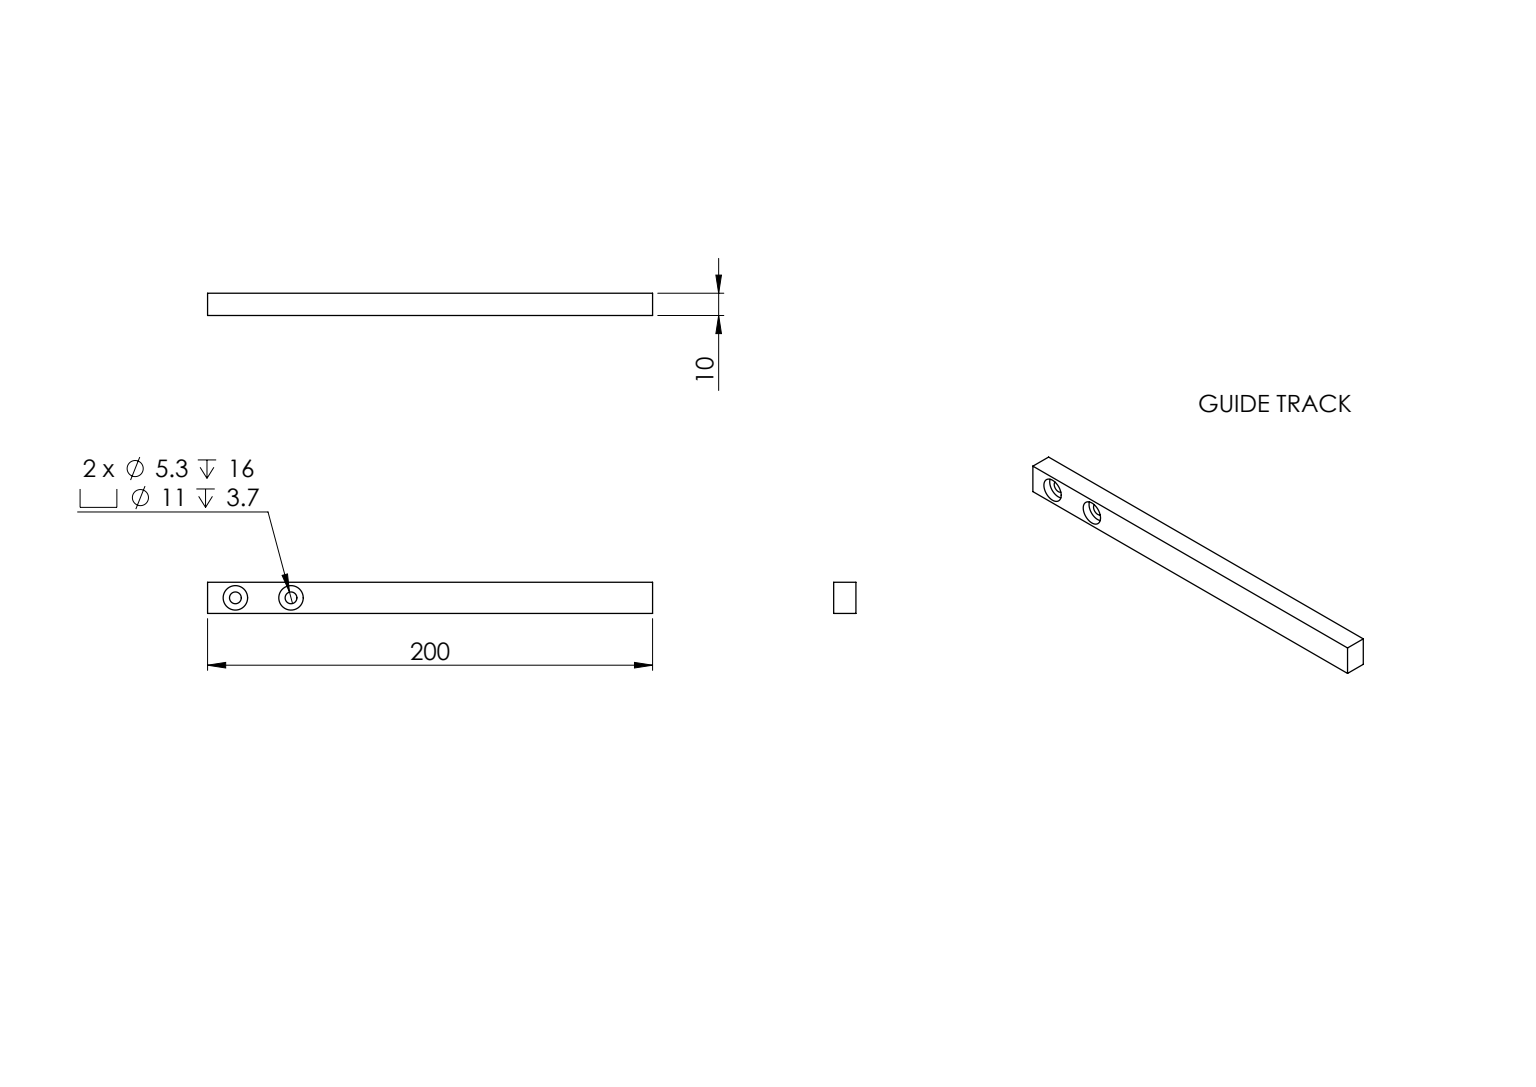
ISO-10303-21;
HEADER;
FILE_DESCRIPTION (('STEP AP214'),
    '1' );
FILE_NAME ('guide track.step',
    '2026-10-27T14:18:53',
    ( '' ),
    ( '' ),
    'SwSTEP 2.0',
    'SolidWorks 2026',
    '' );
FILE_SCHEMA (( 'AUTOMOTIVE_DESIGN' ));
ENDSEC;

DATA;
#9=CIRCLE ( 'NONE', #2713, 2.649999999999999467 ) ;
#10=FACE_OUTER_BOUND ( 'NONE', #5268, .T. ) ;
#20=ADVANCED_FACE ( 'NONE', ( #1293 ), #2022, .F. ) ;
#49=EDGE_LOOP ( 'NONE', ( #4386, #5805, #654, #4968 ) ) ;
#54=CARTESIAN_POINT ( 'NONE',  ( 0.000000000000000000, 0.000000000000000000, 75.00000000000000000 ) ) ;
#60=VERTEX_POINT ( 'NONE', #3659 ) ;
#71=AXIS2_PLACEMENT_3D ( 'NONE', #3867, #5717, #1567 ) ;
#76=CARTESIAN_POINT ( 'NONE',  ( 24.99999999999998224, 6.999999999999985789, 65.00000000000000000 ) ) ;
#84=DIRECTION ( 'NONE',  ( 0.000000000000000000, 0.000000000000000000, 1.000000000000000000 ) ) ;
#91=ADVANCED_FACE ( 'NONE', ( #3214 ), #1319, .F. ) ;
#92=ORIENTED_EDGE ( 'NONE', *, *, #3018, .T. ) ;
#95=DIRECTION ( 'NONE',  ( -0.000000000000000000, -0.000000000000000000, 1.000000000000000000 ) ) ;
#131=EDGE_CURVE ( 'NONE', #60, #666, #9, .T. ) ;
#173=DIRECTION ( 'NONE',  ( -1.000000000000000000, -0.000000000000000000, -0.000000000000000000 ) ) ;
#175=ORIENTED_EDGE ( 'NONE', *, *, #2979, .F. ) ;
#185=AXIS2_PLACEMENT_3D ( 'NONE', #3101, #5825, #5378 ) ;
#220=LINE ( 'NONE', #1177, #2270 ) ;
#235=EDGE_LOOP ( 'NONE', ( #5621, #519 ) ) ;
#242=FACE_BOUND ( 'NONE', #235, .T. ) ;
#271=CARTESIAN_POINT ( 'NONE',  ( 24.99999999999998224, 6.999999999999985789, 75.00000000000000000 ) ) ;
#310=PRESENTATION_STYLE_ASSIGNMENT (( #4469 ) ) ;
#343=CARTESIAN_POINT ( 'NONE',  ( 68.00000000000000000, -1.951563910473909559E-15, 75.00000000000000000 ) ) ;
#346=SHAPE_REPRESENTATION_RELATIONSHIP ( 'NONE' , 'NONE' ,  #2785, #5722 ) ;
#391=DIRECTION ( 'NONE',  ( -0.000000000000000000, -0.000000000000000000, 1.000000000000000000 ) ) ;
#426=CARTESIAN_POINT ( 'NONE',  ( 24.99999999999998224, 6.999999999999985789, 75.00000000000000000 ) ) ;
#438=ORIENTED_EDGE ( 'NONE', *, *, #2529, .F. ) ;
#440=EDGE_LOOP ( 'NONE', ( #5310, #2912, #92, #4963 ) ) ;
#448=EDGE_LOOP ( 'NONE', ( #5357, #973 ) ) ;
#457=DIRECTION ( 'NONE',  ( -0.000000000000000000, -0.000000000000000000, 1.000000000000000000 ) ) ;
#461=EDGE_CURVE ( 'NONE', #5479, #5285, #3793, .T. ) ;
#472=DIRECTION ( 'NONE',  ( 1.000000000000000000, 0.000000000000000000, 0.000000000000000000 ) ) ;
#487=EDGE_LOOP ( 'NONE', ( #1577, #4433, #2223, #5314 ) ) ;
#508=ORIENTED_EDGE ( 'NONE', *, *, #4349, .F. ) ;
#513=DIRECTION ( 'NONE',  ( -0.000000000000000000, -0.000000000000000000, 1.000000000000000000 ) ) ;
#519=ORIENTED_EDGE ( 'NONE', *, *, #2394, .F. ) ;
#566=DIRECTION ( 'NONE',  ( -0.000000000000000000, -0.000000000000000000, 1.000000000000000000 ) ) ;
#599=EDGE_CURVE ( 'NONE', #3899, #5382, #1521, .T. ) ;
#613=CARTESIAN_POINT ( 'NONE',  ( 57.00000000000002132, -1.278008170942866441E-15, 75.00000000000000000 ) ) ;
#615=PRODUCT_DEFINITION_FORMATION_WITH_SPECIFIED_SOURCE ( 'ANY', '', #682, .NOT_KNOWN. ) ;
#638=ORIENTED_EDGE ( 'NONE', *, *, #2527, .F. ) ;
#651=DIRECTION ( 'NONE',  ( -0.000000000000000000, -0.000000000000000000, 1.000000000000000000 ) ) ;
#654=ORIENTED_EDGE ( 'NONE', *, *, #3425, .F. ) ;
#666=VERTEX_POINT ( 'NONE', #3916 ) ;
#667=DIRECTION ( 'NONE',  ( 1.000000000000000000, 0.000000000000000000, 0.000000000000000000 ) ) ;
#681=CARTESIAN_POINT ( 'NONE',  ( 62.50000000000001421, -1.951563910473909559E-15, 75.00000000000000000 ) ) ;
#682=PRODUCT ( 'guide track', 'guide track', '', ( #3710 ) ) ;
#690=DIRECTION ( 'NONE',  ( -0.000000000000000000, -0.000000000000000000, 1.000000000000000000 ) ) ;
#693=CARTESIAN_POINT ( 'NONE',  ( 62.50000000000001421, -1.951563910473909559E-15, 75.00000000000000000 ) ) ;
#709=ORIENTED_EDGE ( 'NONE', *, *, #461, .F. ) ;
#733=ADVANCED_FACE ( 'NONE', ( #10 ), #5052, .F. ) ;
#741=DIRECTION ( 'NONE',  ( 1.000000000000000000, 0.000000000000000000, 0.000000000000000000 ) ) ;
#758=FILL_AREA_STYLE ('',( #4927 ) ) ;
#763=EDGE_CURVE ( 'NONE', #2775, #5479, #5431, .T. ) ;
#778=CYLINDRICAL_SURFACE ( 'NONE', #4471, 2.649999999999999467 ) ;
#790=APPLICATION_CONTEXT ( 'automotive_design' ) ;
#811=CARTESIAN_POINT ( 'NONE',  ( 24.99999999999998224, -7.000000000000006217, 75.00000000000000000 ) ) ;
#818=DIRECTION ( 'NONE',  ( 1.000000000000000000, 0.000000000000000000, 0.000000000000000000 ) ) ;
#823=VERTEX_POINT ( 'NONE', #2303 ) ;
#860=ORIENTED_EDGE ( 'NONE', *, *, #461, .T. ) ;
#868=CARTESIAN_POINT ( 'NONE',  ( 62.50000000000001421, -1.951563910473909559E-15, 75.00000000000000000 ) ) ;
#870=FACE_OUTER_BOUND ( 'NONE', #3951, .T. ) ;
#880=( LENGTH_UNIT ( ) NAMED_UNIT ( * ) SI_UNIT ( .MILLI., .METRE. ) );
#888=VECTOR ( 'NONE', #173, 1000.000000000000000 ) ;
#937=CARTESIAN_POINT ( 'NONE',  ( 24.99999999999998224, 6.999999999999985789, 75.00000000000000000 ) ) ;
#967=DIRECTION ( 'NONE',  ( -0.000000000000000000, -0.000000000000000000, 1.000000000000000000 ) ) ;
#973=ORIENTED_EDGE ( 'NONE', *, *, #1191, .F. ) ;
#994=EDGE_CURVE ( 'NONE', #5382, #3899, #5379, .T. ) ;
#1017=DIRECTION ( 'NONE',  ( -0.000000000000000000, -0.000000000000000000, 1.000000000000000000 ) ) ;
#1026=ORIENTED_EDGE ( 'NONE', *, *, #3647, .T. ) ;
#1062=EDGE_LOOP ( 'NONE', ( #5876, #5322 ) ) ;
#1063=AXIS2_PLACEMENT_3D ( 'NONE', #868, #1807, #4982 ) ;
#1114=ORIENTED_EDGE ( 'NONE', *, *, #763, .F. ) ;
#1126=EDGE_CURVE ( 'NONE', #1974, #666, #220, .T. ) ;
#1130=FACE_OUTER_BOUND ( 'NONE', #1722, .T. ) ;
#1173=AXIS2_PLACEMENT_3D ( 'NONE', #3537, #3080, #741 ) ;
#1177=CARTESIAN_POINT ( 'NONE',  ( 34.85000000000000853, 6.612904002189975595E-15, 75.00000000000000000 ) ) ;
#1178=VECTOR ( 'NONE', #4945, 1000.000000000000000 ) ;
#1179=( GEOMETRIC_REPRESENTATION_CONTEXT ( 3 ) GLOBAL_UNCERTAINTY_ASSIGNED_CONTEXT ( ( #2880 ) ) GLOBAL_UNIT_ASSIGNED_CONTEXT ( ( #3851, #1675, #3797 ) ) REPRESENTATION_CONTEXT ( 'NONE', 'WORKASPACE' ) );
#1191=EDGE_CURVE ( 'NONE', #3398, #3444, #1963, .T. ) ;
#1202=LINE ( 'NONE', #2472, #3651 ) ;
#1207=AXIS2_PLACEMENT_3D ( 'NONE', #3001, #4435, #3875 ) ;
#1216=EDGE_LOOP ( 'NONE', ( #5110, #2401 ) ) ;
#1217=EDGE_LOOP ( 'NONE', ( #4405, #5263, #1114, #1552 ) ) ;
#1223=CARTESIAN_POINT ( 'NONE',  ( 57.00000000000002132, -1.278008170942866441E-15, 71.29999999999999716 ) ) ;
#1233=DIRECTION ( 'NONE',  ( -0.000000000000000000, -0.000000000000000000, 1.000000000000000000 ) ) ;
#1236=ORIENTED_EDGE ( 'NONE', *, *, #2953, .T. ) ;
#1250=CARTESIAN_POINT ( 'NONE',  ( 32.00000000000001421, 6.961928339946971399E-15, 75.00000000000000000 ) ) ;
#1253=DIRECTION ( 'NONE',  ( -0.000000000000000000, -0.000000000000000000, 1.000000000000000000 ) ) ;
#1258=CARTESIAN_POINT ( 'NONE',  ( 37.50000000000000711, 6.288372600415927295E-15, 75.00000000000000000 ) ) ;
#1264=DIRECTION ( 'NONE',  ( 1.000000000000000000, 0.000000000000000000, -0.000000000000000000 ) ) ;
#1289=VERTEX_POINT ( 'NONE', #5943 ) ;
#1293=FACE_OUTER_BOUND ( 'NONE', #440, .T. ) ;
#1303=CLOSED_SHELL ( 'NONE', ( #2062, #3732, #3754, #2960, #5833, #1769, #5035, #91, #1932, #4770, #733, #2348, #5038, #5880, #1455, #20 ) ) ;
#1319=PLANE ( 'NONE',  #3869 ) ;
#1321=DIRECTION ( 'NONE',  ( -1.000000000000000000, 4.770489558936220126E-17, 0.000000000000000000 ) ) ;
#1325=VERTEX_POINT ( 'NONE', #343 ) ;
#1352=DIRECTION ( 'NONE',  ( 1.000000000000000000, 0.000000000000000000, 0.000000000000000000 ) ) ;
#1356=CARTESIAN_POINT ( 'NONE',  ( 62.50000000000001421, -1.951563910473909559E-15, 71.29999999999999716 ) ) ;
#1378=ORIENTED_EDGE ( 'NONE', *, *, #3145, .F. ) ;
#1433=CARTESIAN_POINT ( 'NONE',  ( 62.50000000000001421, -1.951563910473909559E-15, 65.00000000000000000 ) ) ;
#1455=ADVANCED_FACE ( 'NONE', ( #242, #1597 ), #4455, .F. ) ;
#1458=VECTOR ( 'NONE', #690, 1000.000000000000000 ) ;
#1470=FACE_OUTER_BOUND ( 'NONE', #49, .T. ) ;
#1494=ORIENTED_EDGE ( 'NONE', *, *, #3953, .T. ) ;
#1506=CARTESIAN_POINT ( 'NONE',  ( 24.99999999999998224, -7.000000000000006217, 75.00000000000000000 ) ) ;
#1519=ORIENTED_EDGE ( 'NONE', *, *, #2239, .T. ) ;
#1521=CIRCLE ( 'NONE', #185, 5.499999999999991118 ) ;
#1552=ORIENTED_EDGE ( 'NONE', *, *, #4555, .T. ) ;
#1567=DIRECTION ( 'NONE',  ( 1.000000000000000000, 0.000000000000000000, 0.000000000000000000 ) ) ;
#1577=ORIENTED_EDGE ( 'NONE', *, *, #3496, .F. ) ;
#1578=DIRECTION ( 'NONE',  ( 1.000000000000000000, 0.000000000000000000, 0.000000000000000000 ) ) ;
#1583=EDGE_CURVE ( 'NONE', #1856, #2744, #1202, .T. ) ;
#1592=ORIENTED_EDGE ( 'NONE', *, *, #3425, .T. ) ;
#1594=CYLINDRICAL_SURFACE ( 'NONE', #4674, 5.499999999999991118 ) ;
#1597=FACE_OUTER_BOUND ( 'NONE', #4974, .T. ) ;
#1601=DIRECTION ( 'NONE',  ( 1.000000000000000000, 0.000000000000000000, 0.000000000000000000 ) ) ;
#1608=PRODUCT_DEFINITION_CONTEXT ( 'detailed design', #790, 'design' ) ;
#1612=EDGE_CURVE ( 'NONE', #5526, #1289, #5877, .T. ) ;
#1630=LINE ( 'NONE', #5367, #1458 ) ;
#1644=CARTESIAN_POINT ( 'NONE',  ( 37.50000000000000711, 6.288372600415927295E-15, 71.29999999999999716 ) ) ;
#1660=DIRECTION ( 'NONE',  ( 0.000000000000000000, 0.000000000000000000, -1.000000000000000000 ) ) ;
#1661=AXIS2_PLACEMENT_3D ( 'NONE', #2869, #1017, #1352 ) ;
#1669=CIRCLE ( 'NONE', #5920, 2.649999999999999467 ) ;
#1675=( NAMED_UNIT ( * ) PLANE_ANGLE_UNIT ( ) SI_UNIT ( $, .RADIAN. ) );
#1695=FACE_BOUND ( 'NONE', #1062, .T. ) ;
#1703=DIRECTION ( 'NONE',  ( 0.000000000000000000, -1.000000000000000000, 0.000000000000000000 ) ) ;
#1709=CARTESIAN_POINT ( 'NONE',  ( 224.9999999999999716, 6.999999999999985789, 75.00000000000000000 ) ) ;
#1710=DIRECTION ( 'NONE',  ( 0.000000000000000000, 0.000000000000000000, 1.000000000000000000 ) ) ;
#1715=EDGE_CURVE ( 'NONE', #2159, #5534, #4295, .T. ) ;
#1722=EDGE_LOOP ( 'NONE', ( #4931, #1841, #3678, #5341 ) ) ;
#1724=DIRECTION ( 'NONE',  ( -0.000000000000000000, -0.000000000000000000, 1.000000000000000000 ) ) ;
#1769=ADVANCED_FACE ( 'NONE', ( #4980 ), #4547, .F. ) ;
#1792=LINE ( 'NONE', #1506, #2327 ) ;
#1802=CARTESIAN_POINT ( 'NONE',  ( 68.00000000000000000, -1.951563910473909559E-15, 71.29999999999999716 ) ) ;
#1807=DIRECTION ( 'NONE',  ( -0.000000000000000000, -0.000000000000000000, 1.000000000000000000 ) ) ;
#1841=ORIENTED_EDGE ( 'NONE', *, *, #4349, .T. ) ;
#1845=VECTOR ( 'NONE', #566, 1000.000000000000000 ) ;
#1847=CIRCLE ( 'NONE', #1063, 5.499999999999991118 ) ;
#1856=VERTEX_POINT ( 'NONE', #5565 ) ;
#1863=STYLED_ITEM ( 'NONE', ( #310 ), #5722 ) ;
#1864=FACE_BOUND ( 'NONE', #4858, .T. ) ;
#1916=FACE_OUTER_BOUND ( 'NONE', #1217, .T. ) ;
#1932=ADVANCED_FACE ( 'NONE', ( #1864, #5121, #5097 ), #2778, .T. ) ;
#1943=CIRCLE ( 'NONE', #1173, 2.649999999999999467 ) ;
#1944=ORIENTED_EDGE ( 'NONE', *, *, #994, .T. ) ;
#1946=VECTOR ( 'NONE', #4404, 1000.000000000000000 ) ;
#1950=LINE ( 'NONE', #2895, #888 ) ;
#1963=CIRCLE ( 'NONE', #5086, 2.649999999999999467 ) ;
#1971=DIRECTION ( 'NONE',  ( -0.000000000000000000, -0.000000000000000000, 1.000000000000000000 ) ) ;
#1974=VERTEX_POINT ( 'NONE', #4811 ) ;
#2022=CYLINDRICAL_SURFACE ( 'NONE', #1207, 5.499999999999991118 ) ;
#2036=CIRCLE ( 'NONE', #4274, 5.499999999999998224 ) ;
#2056=VECTOR ( 'NONE', #4989, 1000.000000000000000 ) ;
#2062=ADVANCED_FACE ( 'NONE', ( #3377 ), #2099, .F. ) ;
#2069=CARTESIAN_POINT ( 'NONE',  ( 65.15000000000001990, -1.951563910473909559E-15, 71.29999999999999716 ) ) ;
#2099=CYLINDRICAL_SURFACE ( 'NONE', #3855, 5.499999999999991118 ) ;
#2155=( LENGTH_UNIT ( ) NAMED_UNIT ( * ) SI_UNIT ( .MILLI., .METRE. ) );
#2159=VERTEX_POINT ( 'NONE', #1250 ) ;
#2168=CARTESIAN_POINT ( 'NONE',  ( 59.85000000000001563, -1.627032508699861061E-15, 71.29999999999999716 ) ) ;
#2178=DIRECTION ( 'NONE',  ( -0.000000000000000000, -0.000000000000000000, -1.000000000000000000 ) ) ;
#2223=ORIENTED_EDGE ( 'NONE', *, *, #2394, .T. ) ;
#2239=EDGE_CURVE ( 'NONE', #4118, #3289, #5090, .T. ) ;
#2270=VECTOR ( 'NONE', #5287, 1000.000000000000000 ) ;
#2271=DIRECTION ( 'NONE',  ( 1.000000000000000000, 0.000000000000000000, -0.000000000000000000 ) ) ;
#2303=CARTESIAN_POINT ( 'NONE',  ( 32.00000000000000711, 6.961928339946972976E-15, 71.29999999999999716 ) ) ;
#2309=ORIENTED_EDGE ( 'NONE', *, *, #4779, .F. ) ;
#2327=VECTOR ( 'NONE', #2847, 1000.000000000000000 ) ;
#2343=MECHANICAL_DESIGN_GEOMETRIC_PRESENTATION_REPRESENTATION('',(#4482),#1179);
#2348=ADVANCED_FACE ( 'NONE', ( #2980, #4806 ), #3011, .F. ) ;
#2353=LINE ( 'NONE', #3721, #2913 ) ;
#2381=DIRECTION ( 'NONE',  ( -1.000000000000000000, 0.000000000000000000, 0.000000000000000000 ) ) ;
#2394=EDGE_CURVE ( 'NONE', #666, #60, #5522, .T. ) ;
#2401=ORIENTED_EDGE ( 'NONE', *, *, #3250, .T. ) ;
#2406=CARTESIAN_POINT ( 'NONE',  ( 37.50000000000000711, 6.288372600415927295E-15, 75.00000000000000000 ) ) ;
#2413=PRODUCT_DEFINITION ( 'UNKNOWN', '', #615, #1608 ) ;
#2414=AXIS2_PLACEMENT_3D ( 'NONE', #2069, #5674, #4321 ) ;
#2472=CARTESIAN_POINT ( 'NONE',  ( 24.99999999999998224, -7.000000000000006217, 65.00000000000000000 ) ) ;
#2490=DIRECTION ( 'NONE',  ( -0.000000000000000000, -0.000000000000000000, 1.000000000000000000 ) ) ;
#2492=CARTESIAN_POINT ( 'NONE',  ( 37.50000000000000711, 6.288372600415927295E-15, 71.29999999999999716 ) ) ;
#2500=CARTESIAN_POINT ( 'NONE',  ( 24.99999999999998224, -7.000000000000006217, 75.00000000000000000 ) ) ;
#2517=ORIENTED_EDGE ( 'NONE', *, *, #1583, .T. ) ;
#2527=EDGE_CURVE ( 'NONE', #4082, #1856, #5798, .T. ) ;
#2529=EDGE_CURVE ( 'NONE', #823, #5679, #2715, .T. ) ;
#2533=VECTOR ( 'NONE', #1233, 1000.000000000000000 ) ;
#2542=AXIS2_PLACEMENT_3D ( 'NONE', #693, #5309, #1601 ) ;
#2560=DIRECTION ( 'NONE',  ( 1.000000000000000000, 0.000000000000000000, 0.000000000000000000 ) ) ;
#2597=FACE_BOUND ( 'NONE', #1216, .T. ) ;
#2601=EDGE_LOOP ( 'NONE', ( #4126, #5782 ) ) ;
#2605=SURFACE_STYLE_FILL_AREA ( #758 ) ;
#2631=CARTESIAN_POINT ( 'NONE',  ( 43.00000000000000000, 6.288372600415927295E-15, 71.29999999999999716 ) ) ;
#2649=ORIENTED_EDGE ( 'NONE', *, *, #3835, .T. ) ;
#2666=DIRECTION ( 'NONE',  ( 0.000000000000000000, 0.000000000000000000, 1.000000000000000000 ) ) ;
#2687=EDGE_CURVE ( 'NONE', #1289, #3398, #4758, .T. ) ;
#2693=EDGE_CURVE ( 'NONE', #5479, #1856, #1792, .T. ) ;
#2702=CARTESIAN_POINT ( 'NONE',  ( 59.85000000000001563, -1.627032508699861061E-15, 75.00000000000000000 ) ) ;
#2713=AXIS2_PLACEMENT_3D ( 'NONE', #3740, #513, #5589 ) ;
#2715=CIRCLE ( 'NONE', #4957, 5.499999999999998224 ) ;
#2721=DIRECTION ( 'NONE',  ( 1.000000000000000000, 0.000000000000000000, 0.000000000000000000 ) ) ;
#2736=( NAMED_UNIT ( * ) SI_UNIT ( $, .STERADIAN. ) SOLID_ANGLE_UNIT ( ) );
#2744=VERTEX_POINT ( 'NONE', #4309 ) ;
#2745=ORIENTED_EDGE ( 'NONE', *, *, #2687, .T. ) ;
#2766=DIRECTION ( 'NONE',  ( 0.000000000000000000, -1.000000000000000000, 0.000000000000000000 ) ) ;
#2775=VERTEX_POINT ( 'NONE', #4248 ) ;
#2777=DIRECTION ( 'NONE',  ( 0.000000000000000000, -1.000000000000000000, 0.000000000000000000 ) ) ;
#2778=PLANE ( 'NONE',  #4554 ) ;
#2785=SHAPE_REPRESENTATION ( 'guide track', ( #5080 ), #3707 ) ;
#2834=ORIENTED_EDGE ( 'NONE', *, *, #3250, .F. ) ;
#2841=PLANE ( 'NONE',  #4098 ) ;
#2847=DIRECTION ( 'NONE',  ( -0.000000000000000000, -0.000000000000000000, -1.000000000000000000 ) ) ;
#2869=CARTESIAN_POINT ( 'NONE',  ( 62.50000000000001421, -1.951563910473909559E-15, 75.00000000000000000 ) ) ;
#2876=ORIENTED_EDGE ( 'NONE', *, *, #2687, .F. ) ;
#2880=UNCERTAINTY_MEASURE_WITH_UNIT (LENGTH_MEASURE( 1.000000000000000082E-05 ), #3851, 'distance_accuracy_value', 'NONE');
#2895=CARTESIAN_POINT ( 'NONE',  ( 24.99999999999998224, 6.999999999999985789, 75.00000000000000000 ) ) ;
#2912=ORIENTED_EDGE ( 'NONE', *, *, #3322, .F. ) ;
#2913=VECTOR ( 'NONE', #4750, 1000.000000000000000 ) ;
#2937=DIRECTION ( 'NONE',  ( 1.000000000000000000, -4.770489558936219510E-17, 0.000000000000000000 ) ) ;
#2947=UNCERTAINTY_MEASURE_WITH_UNIT (LENGTH_MEASURE( 1.000000000000000082E-05 ), #880, 'distance_accuracy_value', 'NONE');
#2953=EDGE_CURVE ( 'NONE', #1325, #5963, #1847, .T. ) ;
#2960=ADVANCED_FACE ( 'NONE', ( #4150 ), #778, .F. ) ;
#2979=EDGE_CURVE ( 'NONE', #5526, #3444, #3186, .T. ) ;
#2980=FACE_BOUND ( 'NONE', #448, .T. ) ;
#2990=ORIENTED_EDGE ( 'NONE', *, *, #1191, .T. ) ;
#3001=CARTESIAN_POINT ( 'NONE',  ( 37.50000000000000711, 6.288372600415927295E-15, 75.00000000000000000 ) ) ;
#3011=PLANE ( 'NONE',  #2414 ) ;
#3018=EDGE_CURVE ( 'NONE', #5679, #5534, #3602, .T. ) ;
#3032=COLOUR_RGB ( '',0.8941176470588234615, 0.8941176470588234615, 0.8941176470588234615 ) ;
#3080=DIRECTION ( 'NONE',  ( -0.000000000000000000, -0.000000000000000000, 1.000000000000000000 ) ) ;
#3091=ORIENTED_EDGE ( 'NONE', *, *, #1715, .T. ) ;
#3101=CARTESIAN_POINT ( 'NONE',  ( 62.50000000000001421, -1.951563910473909559E-15, 71.29999999999999716 ) ) ;
#3130=MECHANICAL_DESIGN_GEOMETRIC_PRESENTATION_REPRESENTATION('',(#1863),#5837);
#3137=CARTESIAN_POINT ( 'NONE',  ( 62.50000000000001421, -1.951563910473909559E-15, 75.00000000000000000 ) ) ;
#3145=EDGE_CURVE ( 'NONE', #3289, #4082, #2353, .T. ) ;
#3156=AXIS2_PLACEMENT_3D ( 'NONE', #4253, #95, #1578 ) ;
#3183=DIRECTION ( 'NONE',  ( 0.000000000000000000, -0.000000000000000000, -1.000000000000000000 ) ) ;
#3186=LINE ( 'NONE', #4493, #4662 ) ;
#3203=AXIS2_PLACEMENT_3D ( 'NONE', #4351, #1971, #5739 ) ;
#3214=FACE_OUTER_BOUND ( 'NONE', #4629, .T. ) ;
#3219=CARTESIAN_POINT ( 'NONE',  ( 40.15000000000000568, 6.288372600415927295E-15, 65.00000000000000000 ) ) ;
#3230=AXIS2_PLACEMENT_3D ( 'NONE', #5608, #967, #3344 ) ;
#3239=EDGE_LOOP ( 'NONE', ( #1944, #3258 ) ) ;
#3250=EDGE_CURVE ( 'NONE', #1289, #5526, #5343, .T. ) ;
#3258=ORIENTED_EDGE ( 'NONE', *, *, #599, .T. ) ;
#3261=CARTESIAN_POINT ( 'NONE',  ( 224.9999999999999716, 6.999999999999985789, 75.00000000000000000 ) ) ;
#3289=VERTEX_POINT ( 'NONE', #3379 ) ;
#3322=EDGE_CURVE ( 'NONE', #5679, #823, #2036, .T. ) ;
#3333=CYLINDRICAL_SURFACE ( 'NONE', #1661, 5.499999999999991118 ) ;
#3344=DIRECTION ( 'NONE',  ( 1.000000000000000000, 0.000000000000000000, 0.000000000000000000 ) ) ;
#3377=FACE_OUTER_BOUND ( 'NONE', #5364, .T. ) ;
#3379=CARTESIAN_POINT ( 'NONE',  ( 224.9999999999999716, 6.999999999999985789, 65.00000000000000000 ) ) ;
#3389=VECTOR ( 'NONE', #5143, 1000.000000000000000 ) ;
#3398=VERTEX_POINT ( 'NONE', #2168 ) ;
#3420=CARTESIAN_POINT ( 'NONE',  ( 40.15000000000000568, 6.288372600415927295E-15, 71.29999999999999716 ) ) ;
#3425=EDGE_CURVE ( 'NONE', #5285, #4118, #3536, .T. ) ;
#3430=ORIENTED_EDGE ( 'NONE', *, *, #3018, .F. ) ;
#3444=VERTEX_POINT ( 'NONE', #5030 ) ;
#3493=DIRECTION ( 'NONE',  ( 1.000000000000000000, 0.000000000000000000, 0.000000000000000000 ) ) ;
#3496=EDGE_CURVE ( 'NONE', #1974, #5044, #4864, .T. ) ;
#3527=CARTESIAN_POINT ( 'NONE',  ( 0.000000000000000000, 0.000000000000000000, 0.000000000000000000 ) ) ;
#3536=LINE ( 'NONE', #1709, #5441 ) ;
#3537=CARTESIAN_POINT ( 'NONE',  ( 62.50000000000001421, -1.951563910473909559E-15, 71.29999999999999716 ) ) ;
#3564=DIRECTION ( 'NONE',  ( 1.000000000000000000, 0.000000000000000000, 0.000000000000000000 ) ) ;
#3571=LINE ( 'NONE', #5396, #1178 ) ;
#3578=EDGE_LOOP ( 'NONE', ( #5516, #860, #1592, #2649 ) ) ;
#3602=LINE ( 'NONE', #5012, #4960 ) ;
#3604=PLANE ( 'NONE',  #5718 ) ;
#3616=( NAMED_UNIT ( * ) PLANE_ANGLE_UNIT ( ) SI_UNIT ( $, .RADIAN. ) );
#3627=DIRECTION ( 'NONE',  ( 0.000000000000000000, 0.000000000000000000, 1.000000000000000000 ) ) ;
#3647=EDGE_CURVE ( 'NONE', #5382, #1325, #1630, .T. ) ;
#3651=VECTOR ( 'NONE', #2937, 1000.000000000000000 ) ;
#3659=CARTESIAN_POINT ( 'NONE',  ( 40.15000000000000568, 6.288372600415927295E-15, 71.29999999999999716 ) ) ;
#3663=DIRECTION ( 'NONE',  ( -0.000000000000000000, -0.000000000000000000, 1.000000000000000000 ) ) ;
#3678=ORIENTED_EDGE ( 'NONE', *, *, #4602, .T. ) ;
#3707=( GEOMETRIC_REPRESENTATION_CONTEXT ( 3 ) GLOBAL_UNCERTAINTY_ASSIGNED_CONTEXT ( ( #4829 ) ) GLOBAL_UNIT_ASSIGNED_CONTEXT ( ( #2155, #5377, #3943 ) ) REPRESENTATION_CONTEXT ( 'NONE', 'WORKASPACE' ) );
#3710=PRODUCT_CONTEXT ( 'NONE', #4520, 'mechanical' ) ;
#3714=CARTESIAN_POINT ( 'NONE',  ( 224.9999999999999716, 6.999999999999985789, 75.00000000000000000 ) ) ;
#3721=CARTESIAN_POINT ( 'NONE',  ( 24.99999999999998224, 6.999999999999985789, 65.00000000000000000 ) ) ;
#3732=ADVANCED_FACE ( 'NONE', ( #3897 ), #4751, .F. ) ;
#3740=CARTESIAN_POINT ( 'NONE',  ( 37.50000000000000711, 6.288372600415927295E-15, 71.29999999999999716 ) ) ;
#3754=ADVANCED_FACE ( 'NONE', ( #1130 ), #1594, .F. ) ;
#3770=PRODUCT_DEFINITION_SHAPE ( 'NONE', 'NONE',  #2413 ) ;
#3793=LINE ( 'NONE', #5218, #4326 ) ;
#3797=( NAMED_UNIT ( * ) SI_UNIT ( $, .STERADIAN. ) SOLID_ANGLE_UNIT ( ) );
#3835=EDGE_CURVE ( 'NONE', #4118, #2775, #1950, .T. ) ;
#3840=CARTESIAN_POINT ( 'NONE',  ( 43.00000000000000000, 6.288372600415927295E-15, 75.00000000000000000 ) ) ;
#3851=( LENGTH_UNIT ( ) NAMED_UNIT ( * ) SI_UNIT ( .MILLI., .METRE. ) );
#3855=AXIS2_PLACEMENT_3D ( 'NONE', #3950, #2490, #4299 ) ;
#3867=CARTESIAN_POINT ( 'NONE',  ( 62.50000000000001421, -1.951563910473909559E-15, 65.00000000000000000 ) ) ;
#3869=AXIS2_PLACEMENT_3D ( 'NONE', #4663, #2777, #3183 ) ;
#3875=DIRECTION ( 'NONE',  ( 1.000000000000000000, 0.000000000000000000, 0.000000000000000000 ) ) ;
#3877=VECTOR ( 'NONE', #1703, 1000.000000000000000 ) ;
#3886=AXIS2_PLACEMENT_3D ( 'NONE', #2406, #5748, #4726 ) ;
#3897=FACE_OUTER_BOUND ( 'NONE', #487, .T. ) ;
#3899=VERTEX_POINT ( 'NONE', #1223 ) ;
#3916=CARTESIAN_POINT ( 'NONE',  ( 34.85000000000000853, 6.612904002189975595E-15, 71.29999999999999716 ) ) ;
#3922=ORIENTED_EDGE ( 'NONE', *, *, #5615, .F. ) ;
#3942=EDGE_CURVE ( 'NONE', #5044, #1974, #1669, .T. ) ;
#3943=( NAMED_UNIT ( * ) SI_UNIT ( $, .STERADIAN. ) SOLID_ANGLE_UNIT ( ) );
#3950=CARTESIAN_POINT ( 'NONE',  ( 37.50000000000000711, 6.288372600415927295E-15, 75.00000000000000000 ) ) ;
#3951=EDGE_LOOP ( 'NONE', ( #638, #1378, #3922, #3964 ) ) ;
#3953=EDGE_CURVE ( 'NONE', #3444, #3398, #1943, .T. ) ;
#3964=ORIENTED_EDGE ( 'NONE', *, *, #1583, .F. ) ;
#3973=EDGE_CURVE ( 'NONE', #823, #2159, #5412, .T. ) ;
#3994=AXIS2_PLACEMENT_3D ( 'NONE', #3137, #457, #4597 ) ;
#3999=DIRECTION ( 'NONE',  ( -1.000000000000000000, 0.000000000000000000, -0.000000000000000000 ) ) ;
#4008=CARTESIAN_POINT ( 'NONE',  ( 37.50000000000000711, 6.288372600415927295E-15, 75.00000000000000000 ) ) ;
#4011=DIRECTION ( 'NONE',  ( -0.000000000000000000, -0.000000000000000000, 1.000000000000000000 ) ) ;
#4042=CARTESIAN_POINT ( 'NONE',  ( 37.50000000000000711, 6.288372600415927295E-15, 65.00000000000000000 ) ) ;
#4043=CARTESIAN_POINT ( 'NONE',  ( 32.00000000000001421, 6.961928339946971399E-15, 75.00000000000000000 ) ) ;
#4082=VERTEX_POINT ( 'NONE', #76 ) ;
#4089=CARTESIAN_POINT ( 'NONE',  ( 224.9999999999999716, -7.000000000000015987, 75.00000000000000000 ) ) ;
#4091=AXIS2_PLACEMENT_3D ( 'NONE', #426, #2271, #5514 ) ;
#4098=AXIS2_PLACEMENT_3D ( 'NONE', #4701, #2381, #84 ) ;
#4111=EDGE_LOOP ( 'NONE', ( #4680, #5499, #5024, #5569 ) ) ;
#4118=VERTEX_POINT ( 'NONE', #3714 ) ;
#4121=DIRECTION ( 'NONE',  ( 1.000000000000000000, 0.000000000000000000, 0.000000000000000000 ) ) ;
#4126=ORIENTED_EDGE ( 'NONE', *, *, #2953, .F. ) ;
#4150=FACE_OUTER_BOUND ( 'NONE', #5462, .T. ) ;
#4191=LINE ( 'NONE', #271, #1946 ) ;
#4206=MANIFOLD_SOLID_BREP ( 'CBORE for M5 Pan Head Screw1', #1303 ) ;
#4236=DIRECTION ( 'NONE',  ( 1.000000000000000000, 0.000000000000000000, -0.000000000000000000 ) ) ;
#4248=CARTESIAN_POINT ( 'NONE',  ( 24.99999999999998224, 6.999999999999985789, 75.00000000000000000 ) ) ;
#4253=CARTESIAN_POINT ( 'NONE',  ( 62.50000000000001421, -1.951563910473909559E-15, 71.29999999999999716 ) ) ;
#4274=AXIS2_PLACEMENT_3D ( 'NONE', #2492, #651, #2560 ) ;
#4295=CIRCLE ( 'NONE', #4881, 5.499999999999991118 ) ;
#4299=DIRECTION ( 'NONE',  ( 1.000000000000000000, 0.000000000000000000, 0.000000000000000000 ) ) ;
#4309=CARTESIAN_POINT ( 'NONE',  ( 224.9999999999999716, -7.000000000000015987, 65.00000000000000000 ) ) ;
#4321=DIRECTION ( 'NONE',  ( -1.000000000000000000, 0.000000000000000000, -0.000000000000000000 ) ) ;
#4325=EDGE_LOOP ( 'NONE', ( #508, #5594, #1026, #1236 ) ) ;
#4326=VECTOR ( 'NONE', #4774, 1000.000000000000000 ) ;
#4348=SURFACE_SIDE_STYLE ('',( #2605 ) ) ;
#4349=EDGE_CURVE ( 'NONE', #3899, #5963, #5049, .T. ) ;
#4351=CARTESIAN_POINT ( 'NONE',  ( 37.50000000000000711, 6.288372600415927295E-15, 71.29999999999999716 ) ) ;
#4377=AXIS2_PLACEMENT_3D ( 'NONE', #4042, #3627, #3564 ) ;
#4386=ORIENTED_EDGE ( 'NONE', *, *, #5615, .T. ) ;
#4404=DIRECTION ( 'NONE',  ( -0.000000000000000000, -0.000000000000000000, -1.000000000000000000 ) ) ;
#4405=ORIENTED_EDGE ( 'NONE', *, *, #2527, .T. ) ;
#4406=EDGE_CURVE ( 'NONE', #5534, #2159, #5832, .T. ) ;
#4433=ORIENTED_EDGE ( 'NONE', *, *, #1126, .T. ) ;
#4435=DIRECTION ( 'NONE',  ( -0.000000000000000000, -0.000000000000000000, 1.000000000000000000 ) ) ;
#4455=PLANE ( 'NONE',  #4532 ) ;
#4469=SURFACE_STYLE_USAGE ( .BOTH. , #4348 ) ;
#4471=AXIS2_PLACEMENT_3D ( 'NONE', #5418, #5454, #2721 ) ;
#4482=STYLED_ITEM('',(#6006),#4206);
#4488=VECTOR ( 'NONE', #2766, 1000.000000000000000 ) ;
#4493=CARTESIAN_POINT ( 'NONE',  ( 65.15000000000001990, -1.951563910473909559E-15, 75.00000000000000000 ) ) ;
#4519=DIRECTION ( 'NONE',  ( 4.770489558936220126E-17, 1.000000000000000000, -0.000000000000000000 ) ) ;
#4520=APPLICATION_CONTEXT ( 'automotive_design' ) ;
#4522=CARTESIAN_POINT ( 'NONE',  ( 40.15000000000000568, 6.288372600415927295E-15, 75.00000000000000000 ) ) ;
#4529=ORIENTED_EDGE ( 'NONE', *, *, #4406, .F. ) ;
#4532=AXIS2_PLACEMENT_3D ( 'NONE', #3420, #1660, #3999 ) ;
#4547=PLANE ( 'NONE',  #5040 ) ;
#4551=EDGE_LOOP ( 'NONE', ( #2517, #2309, #709, #5776 ) ) ;
#4554=AXIS2_PLACEMENT_3D ( 'NONE', #54, #5590, #4236 ) ;
#4555=EDGE_CURVE ( 'NONE', #2775, #4082, #4191, .T. ) ;
#4571=CIRCLE ( 'NONE', #2542, 5.499999999999991118 ) ;
#4580=PLANE ( 'NONE',  #4091 ) ;
#4597=DIRECTION ( 'NONE',  ( 1.000000000000000000, 0.000000000000000000, 0.000000000000000000 ) ) ;
#4602=EDGE_CURVE ( 'NONE', #5963, #1325, #4571, .T. ) ;
#4629=EDGE_LOOP ( 'NONE', ( #5867, #5119, #4904, #1519 ) ) ;
#4636=DIRECTION ( 'NONE',  ( 0.000000000000000000, 0.000000000000000000, 1.000000000000000000 ) ) ;
#4651=CYLINDRICAL_SURFACE ( 'NONE', #3230, 2.649999999999999467 ) ;
#4662=VECTOR ( 'NONE', #3663, 1000.000000000000000 ) ;
#4663=CARTESIAN_POINT ( 'NONE',  ( 24.99999999999998224, 6.999999999999985789, 75.00000000000000000 ) ) ;
#4674=AXIS2_PLACEMENT_3D ( 'NONE', #681, #5271, #4815 ) ;
#4680=ORIENTED_EDGE ( 'NONE', *, *, #1126, .F. ) ;
#4701=CARTESIAN_POINT ( 'NONE',  ( 224.9999999999999716, 6.999999999999985789, 75.00000000000000000 ) ) ;
#4708=ORIENTED_EDGE ( 'NONE', *, *, #2529, .T. ) ;
#4720=ORIENTED_EDGE ( 'NONE', *, *, #1715, .F. ) ;
#4726=DIRECTION ( 'NONE',  ( 1.000000000000000000, 0.000000000000000000, 0.000000000000000000 ) ) ;
#4750=DIRECTION ( 'NONE',  ( -1.000000000000000000, -0.000000000000000000, -0.000000000000000000 ) ) ;
#4751=CYLINDRICAL_SURFACE ( 'NONE', #3886, 2.649999999999999467 ) ;
#4758=LINE ( 'NONE', #2702, #1845 ) ;
#4770=ADVANCED_FACE ( 'NONE', ( #1695, #2597, #870 ), #3604, .F. ) ;
#4774=DIRECTION ( 'NONE',  ( 1.000000000000000000, -4.770489558936219510E-17, 0.000000000000000000 ) ) ;
#4779=EDGE_CURVE ( 'NONE', #5285, #2744, #5458, .T. ) ;
#4806=FACE_OUTER_BOUND ( 'NONE', #3239, .T. ) ;
#4811=CARTESIAN_POINT ( 'NONE',  ( 34.85000000000000853, 6.612904002189975595E-15, 65.00000000000000000 ) ) ;
#4815=DIRECTION ( 'NONE',  ( 1.000000000000000000, 0.000000000000000000, 0.000000000000000000 ) ) ;
#4829=UNCERTAINTY_MEASURE_WITH_UNIT (LENGTH_MEASURE( 1.000000000000000082E-05 ), #2155, 'distance_accuracy_value', 'NONE');
#4831=DIRECTION ( 'NONE',  ( 0.000000000000000000, 0.000000000000000000, 1.000000000000000000 ) ) ;
#4839=ORIENTED_EDGE ( 'NONE', *, *, #2979, .T. ) ;
#4858=EDGE_LOOP ( 'NONE', ( #4529, #4720 ) ) ;
#4864=CIRCLE ( 'NONE', #4377, 2.649999999999999467 ) ;
#4881=AXIS2_PLACEMENT_3D ( 'NONE', #1258, #5417, #4121 ) ;
#4904=ORIENTED_EDGE ( 'NONE', *, *, #3835, .F. ) ;
#4927=FILL_AREA_STYLE_COLOUR ( '', #3032 ) ;
#4930=CARTESIAN_POINT ( 'NONE',  ( 24.99999999999998224, 6.999999999999985789, 65.00000000000000000 ) ) ;
#4931=ORIENTED_EDGE ( 'NONE', *, *, #599, .F. ) ;
#4945=DIRECTION ( 'NONE',  ( -0.000000000000000000, 1.000000000000000000, -0.000000000000000000 ) ) ;
#4946=CARTESIAN_POINT ( 'NONE',  ( 0.000000000000000000, 0.000000000000000000, 65.00000000000000000 ) ) ;
#4957=AXIS2_PLACEMENT_3D ( 'NONE', #1644, #4011, #3493 ) ;
#4960=VECTOR ( 'NONE', #391, 1000.000000000000000 ) ;
#4963=ORIENTED_EDGE ( 'NONE', *, *, #4406, .T. ) ;
#4968=ORIENTED_EDGE ( 'NONE', *, *, #4779, .T. ) ;
#4974=EDGE_LOOP ( 'NONE', ( #5650, #4708 ) ) ;
#4976=ORIENTED_EDGE ( 'NONE', *, *, #1612, .F. ) ;
#4980=FACE_OUTER_BOUND ( 'NONE', #4551, .T. ) ;
#4982=DIRECTION ( 'NONE',  ( 1.000000000000000000, 0.000000000000000000, 0.000000000000000000 ) ) ;
#4989=DIRECTION ( 'NONE',  ( -0.000000000000000000, -0.000000000000000000, 1.000000000000000000 ) ) ;
#5004=DIRECTION ( 'NONE',  ( -0.000000000000000000, 1.000000000000000000, -0.000000000000000000 ) ) ;
#5007=CARTESIAN_POINT ( 'NONE',  ( 224.9999999999999716, -7.000000000000015987, 75.00000000000000000 ) ) ;
#5012=CARTESIAN_POINT ( 'NONE',  ( 43.00000000000000000, 6.288372600415927295E-15, 75.00000000000000000 ) ) ;
#5024=ORIENTED_EDGE ( 'NONE', *, *, #5647, .T. ) ;
#5030=CARTESIAN_POINT ( 'NONE',  ( 65.15000000000001990, -1.951563910473909559E-15, 71.29999999999999716 ) ) ;
#5035=ADVANCED_FACE ( 'NONE', ( #1470 ), #2841, .F. ) ;
#5038=ADVANCED_FACE ( 'NONE', ( #5625 ), #3333, .F. ) ;
#5040=AXIS2_PLACEMENT_3D ( 'NONE', #811, #4519, #1321 ) ;
#5044=VERTEX_POINT ( 'NONE', #3219 ) ;
#5049=LINE ( 'NONE', #5948, #2056 ) ;
#5052=CYLINDRICAL_SURFACE ( 'NONE', #3994, 2.649999999999999467 ) ;
#5059=AXIS2_PLACEMENT_3D ( 'NONE', #1433, #4636, #472 ) ;
#5070=VECTOR ( 'NONE', #1253, 1000.000000000000000 ) ;
#5080=AXIS2_PLACEMENT_3D ( 'NONE', #3527, #4831, #667 ) ;
#5086=AXIS2_PLACEMENT_3D ( 'NONE', #1356, #1724, #818 ) ;
#5090=LINE ( 'NONE', #3261, #3389 ) ;
#5097=FACE_OUTER_BOUND ( 'NONE', #3578, .T. ) ;
#5110=ORIENTED_EDGE ( 'NONE', *, *, #1612, .T. ) ;
#5119=ORIENTED_EDGE ( 'NONE', *, *, #4555, .F. ) ;
#5121=FACE_BOUND ( 'NONE', #2601, .T. ) ;
#5136=FACE_OUTER_BOUND ( 'NONE', #4111, .T. ) ;
#5143=DIRECTION ( 'NONE',  ( -0.000000000000000000, -0.000000000000000000, -1.000000000000000000 ) ) ;
#5161=DIRECTION ( 'NONE',  ( 1.000000000000000000, 0.000000000000000000, 0.000000000000000000 ) ) ;
#5218=CARTESIAN_POINT ( 'NONE',  ( 24.99999999999998224, -7.000000000000006217, 75.00000000000000000 ) ) ;
#5263=ORIENTED_EDGE ( 'NONE', *, *, #2693, .F. ) ;
#5268=EDGE_LOOP ( 'NONE', ( #2876, #4976, #4839, #1494 ) ) ;
#5271=DIRECTION ( 'NONE',  ( -0.000000000000000000, -0.000000000000000000, 1.000000000000000000 ) ) ;
#5285=VERTEX_POINT ( 'NONE', #5007 ) ;
#5287=DIRECTION ( 'NONE',  ( -0.000000000000000000, -0.000000000000000000, 1.000000000000000000 ) ) ;
#5309=DIRECTION ( 'NONE',  ( -0.000000000000000000, -0.000000000000000000, 1.000000000000000000 ) ) ;
#5310=ORIENTED_EDGE ( 'NONE', *, *, #3973, .F. ) ;
#5314=ORIENTED_EDGE ( 'NONE', *, *, #5647, .F. ) ;
#5322=ORIENTED_EDGE ( 'NONE', *, *, #3496, .T. ) ;
#5341=ORIENTED_EDGE ( 'NONE', *, *, #3647, .F. ) ;
#5343=CIRCLE ( 'NONE', #5059, 2.649999999999999467 ) ;
#5357=ORIENTED_EDGE ( 'NONE', *, *, #3953, .F. ) ;
#5364=EDGE_LOOP ( 'NONE', ( #438, #5563, #3091, #3430 ) ) ;
#5367=CARTESIAN_POINT ( 'NONE',  ( 68.00000000000000000, -1.951563910473909559E-15, 75.00000000000000000 ) ) ;
#5377=( NAMED_UNIT ( * ) PLANE_ANGLE_UNIT ( ) SI_UNIT ( $, .RADIAN. ) );
#5378=DIRECTION ( 'NONE',  ( 1.000000000000000000, 0.000000000000000000, 0.000000000000000000 ) ) ;
#5379=CIRCLE ( 'NONE', #3156, 5.499999999999991118 ) ;
#5382=VERTEX_POINT ( 'NONE', #1802 ) ;
#5387=DIRECTION ( 'NONE',  ( 1.000000000000000000, 0.000000000000000000, 0.000000000000000000 ) ) ;
#5396=CARTESIAN_POINT ( 'NONE',  ( 224.9999999999999716, 6.999999999999985789, 65.00000000000000000 ) ) ;
#5412=LINE ( 'NONE', #4043, #5070 ) ;
#5417=DIRECTION ( 'NONE',  ( -0.000000000000000000, -0.000000000000000000, 1.000000000000000000 ) ) ;
#5418=CARTESIAN_POINT ( 'NONE',  ( 62.50000000000001421, -1.951563910473909559E-15, 75.00000000000000000 ) ) ;
#5431=LINE ( 'NONE', #937, #4488 ) ;
#5432=VECTOR ( 'NONE', #2178, 1000.000000000000000 ) ;
#5441=VECTOR ( 'NONE', #5004, 1000.000000000000000 ) ;
#5454=DIRECTION ( 'NONE',  ( -0.000000000000000000, -0.000000000000000000, 1.000000000000000000 ) ) ;
#5458=LINE ( 'NONE', #4089, #5432 ) ;
#5462=EDGE_LOOP ( 'NONE', ( #2834, #2745, #2990, #175 ) ) ;
#5479=VERTEX_POINT ( 'NONE', #2500 ) ;
#5486=LINE ( 'NONE', #4522, #2533 ) ;
#5499=ORIENTED_EDGE ( 'NONE', *, *, #3942, .F. ) ;
#5514=DIRECTION ( 'NONE',  ( -0.000000000000000000, 0.000000000000000000, -1.000000000000000000 ) ) ;
#5516=ORIENTED_EDGE ( 'NONE', *, *, #763, .T. ) ;
#5522=CIRCLE ( 'NONE', #3203, 2.649999999999999467 ) ;
#5526=VERTEX_POINT ( 'NONE', #5663 ) ;
#5534=VERTEX_POINT ( 'NONE', #3840 ) ;
#5558=SHAPE_DEFINITION_REPRESENTATION ( #3770, #2785 ) ;
#5563=ORIENTED_EDGE ( 'NONE', *, *, #3973, .T. ) ;
#5565=CARTESIAN_POINT ( 'NONE',  ( 24.99999999999998224, -7.000000000000006217, 65.00000000000000000 ) ) ;
#5569=ORIENTED_EDGE ( 'NONE', *, *, #131, .T. ) ;
#5589=DIRECTION ( 'NONE',  ( 1.000000000000000000, 0.000000000000000000, 0.000000000000000000 ) ) ;
#5590=DIRECTION ( 'NONE',  ( 0.000000000000000000, 0.000000000000000000, 1.000000000000000000 ) ) ;
#5594=ORIENTED_EDGE ( 'NONE', *, *, #994, .F. ) ;
#5608=CARTESIAN_POINT ( 'NONE',  ( 37.50000000000000711, 6.288372600415927295E-15, 75.00000000000000000 ) ) ;
#5615=EDGE_CURVE ( 'NONE', #2744, #3289, #3571, .T. ) ;
#5621=ORIENTED_EDGE ( 'NONE', *, *, #131, .F. ) ;
#5625=FACE_OUTER_BOUND ( 'NONE', #4325, .T. ) ;
#5633=AXIS2_PLACEMENT_3D ( 'NONE', #4008, #5856, #5161 ) ;
#5647=EDGE_CURVE ( 'NONE', #5044, #60, #5486, .T. ) ;
#5650=ORIENTED_EDGE ( 'NONE', *, *, #3322, .T. ) ;
#5663=CARTESIAN_POINT ( 'NONE',  ( 65.15000000000001990, -1.951563910473909559E-15, 65.00000000000000000 ) ) ;
#5674=DIRECTION ( 'NONE',  ( 0.000000000000000000, 0.000000000000000000, -1.000000000000000000 ) ) ;
#5679=VERTEX_POINT ( 'NONE', #2631 ) ;
#5717=DIRECTION ( 'NONE',  ( 0.000000000000000000, 0.000000000000000000, 1.000000000000000000 ) ) ;
#5718=AXIS2_PLACEMENT_3D ( 'NONE', #4946, #2666, #1264 ) ;
#5722=ADVANCED_BREP_SHAPE_REPRESENTATION ( '', ( #4206, #5080 ), #3707 ) ;
#5739=DIRECTION ( 'NONE',  ( 1.000000000000000000, 0.000000000000000000, 0.000000000000000000 ) ) ;
#5748=DIRECTION ( 'NONE',  ( -0.000000000000000000, -0.000000000000000000, 1.000000000000000000 ) ) ;
#5776=ORIENTED_EDGE ( 'NONE', *, *, #2693, .T. ) ;
#5782=ORIENTED_EDGE ( 'NONE', *, *, #4602, .F. ) ;
#5798=LINE ( 'NONE', #4930, #3877 ) ;
#5805=ORIENTED_EDGE ( 'NONE', *, *, #2239, .F. ) ;
#5825=DIRECTION ( 'NONE',  ( -0.000000000000000000, -0.000000000000000000, 1.000000000000000000 ) ) ;
#5832=CIRCLE ( 'NONE', #5633, 5.499999999999991118 ) ;
#5833=ADVANCED_FACE ( 'NONE', ( #1916 ), #4580, .F. ) ;
#5837=( GEOMETRIC_REPRESENTATION_CONTEXT ( 3 ) GLOBAL_UNCERTAINTY_ASSIGNED_CONTEXT ( ( #2947 ) ) GLOBAL_UNIT_ASSIGNED_CONTEXT ( ( #880, #3616, #2736 ) ) REPRESENTATION_CONTEXT ( 'NONE', 'WORKASPACE' ) );
#5841=CARTESIAN_POINT ( 'NONE',  ( 37.50000000000000711, 6.288372600415927295E-15, 65.00000000000000000 ) ) ;
#5856=DIRECTION ( 'NONE',  ( -0.000000000000000000, -0.000000000000000000, 1.000000000000000000 ) ) ;
#5867=ORIENTED_EDGE ( 'NONE', *, *, #3145, .T. ) ;
#5876=ORIENTED_EDGE ( 'NONE', *, *, #3942, .T. ) ;
#5877=CIRCLE ( 'NONE', #71, 2.649999999999999467 ) ;
#5880=ADVANCED_FACE ( 'NONE', ( #5136 ), #4651, .F. ) ;
#5920=AXIS2_PLACEMENT_3D ( 'NONE', #5841, #1710, #5387 ) ;
#5943=CARTESIAN_POINT ( 'NONE',  ( 59.85000000000001563, -1.627032508699861061E-15, 65.00000000000000000 ) ) ;
#5948=CARTESIAN_POINT ( 'NONE',  ( 57.00000000000002132, -1.278008170942866441E-15, 75.00000000000000000 ) ) ;
#5963=VERTEX_POINT ( 'NONE', #613 ) ;
#6000=COLOUR_RGB('Light Blue',0.38,0.62,0.78);
#6001=FILL_AREA_STYLE_COLOUR('',#6000);
#6002=FILL_AREA_STYLE('',(#6001));
#6003=SURFACE_STYLE_FILL_AREA(#6002);
#6004=SURFACE_SIDE_STYLE('',(#6003));
#6005=SURFACE_STYLE_USAGE(.BOTH.,#6004);
#6006=PRESENTATION_STYLE_ASSIGNMENT((#6005));
ENDSEC;
END-ISO-10303-21;
